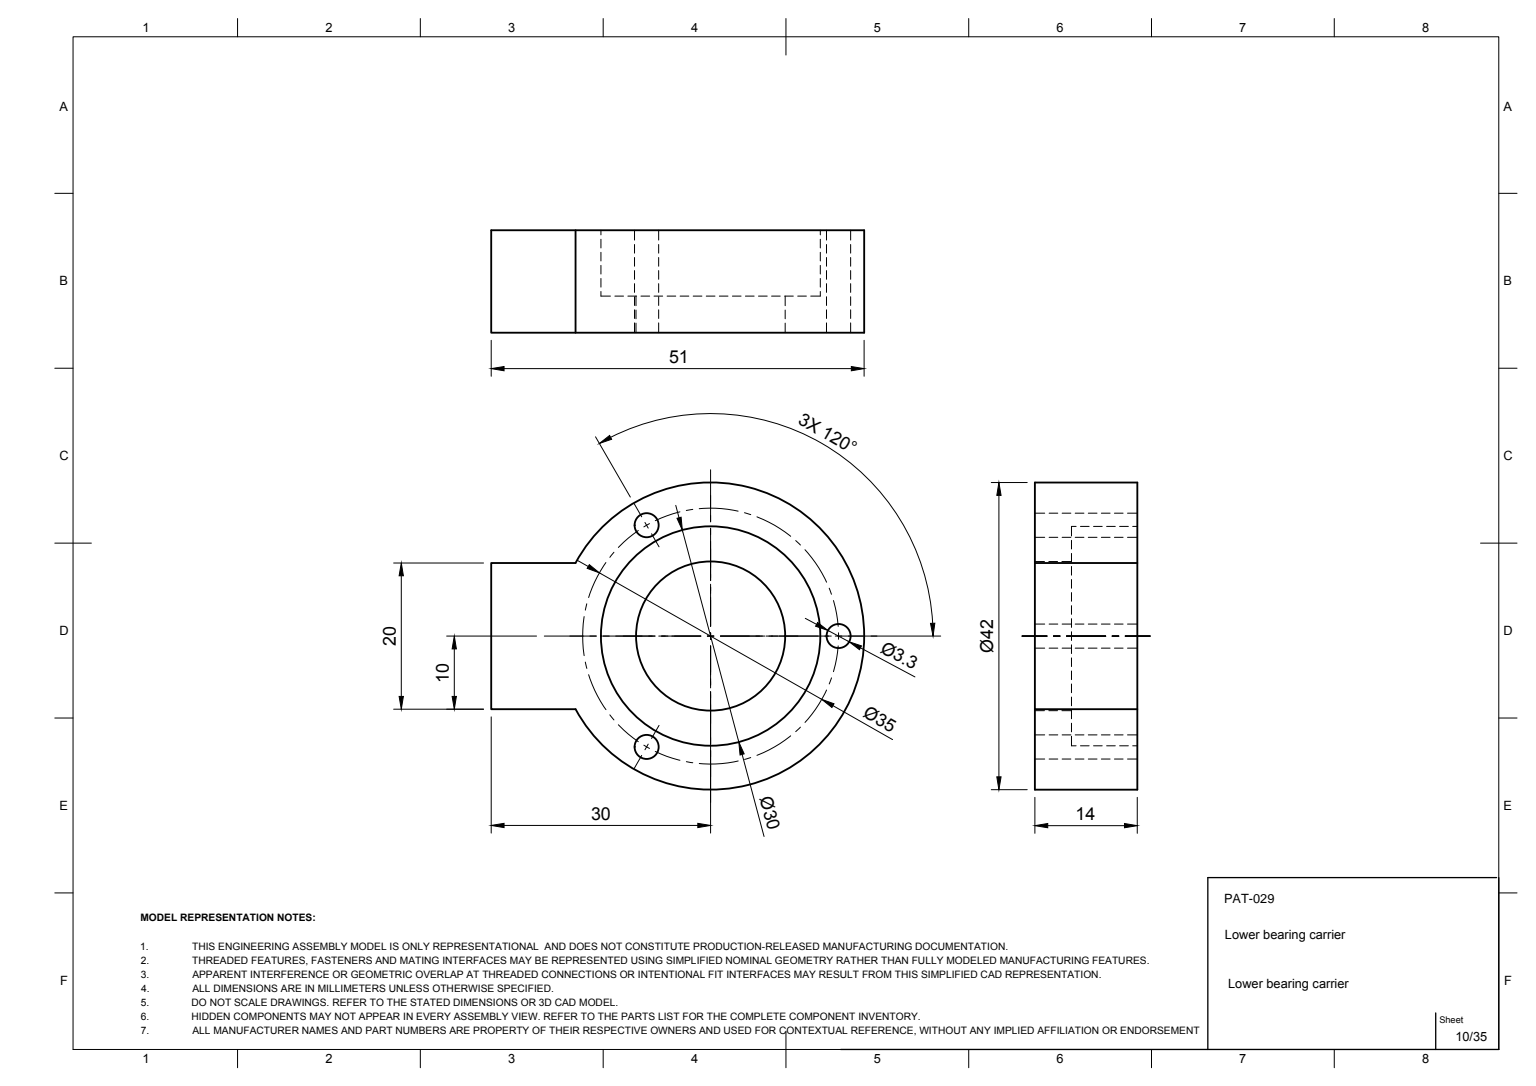
ISO-10303-21;
HEADER;
/* Generated by software containing ST-Developer
 * from STEP Tools, Inc. (www.steptools.com) 
 */

FILE_DESCRIPTION(
/* description */ ('Door-style hinge test fixture with detent'),
/* implementation_level */ '2;1');

FILE_NAME(
/* name */ 'Lower bearing carrier.step',
/* time_stamp */ '2026-10-28T03:24:57-07:00',
/* author */ (''),
/* organization */ (''),
/* preprocessor_version */ 'ST-DEVELOPER v20.2',
/* originating_system */ 'Autodesk Translation Framework v15.17.0.0',
/* authorisation */ '');

FILE_SCHEMA (('AUTOMOTIVE_DESIGN { 1 0 10303 214 3 1 1 }'));
ENDSEC;

DATA;
#10=MECHANICAL_DESIGN_GEOMETRIC_PRESENTATION_REPRESENTATION('',(#328),#9813);
#265=SHAPE_REPRESENTATION_RELATIONSHIP('SRR','None',#9942,#296);
#296=ADVANCED_BREP_SHAPE_REPRESENTATION('',(#368),#9785);
#328=STYLED_ITEM('',(#10183),#368);
#368=MANIFOLD_SOLID_BREP('Body1',#4759);
#423=FACE_BOUND('',#1025,.T.);
#424=FACE_BOUND('',#1028,.T.);
#425=FACE_BOUND('',#1029,.T.);
#426=FACE_BOUND('',#1030,.T.);
#427=FACE_BOUND('',#1031,.T.);
#428=FACE_BOUND('',#1037,.T.);
#429=FACE_BOUND('',#1038,.T.);
#430=FACE_BOUND('',#1039,.T.);
#431=FACE_BOUND('',#1040,.T.);
#536=PLANE('',#5230);
#537=PLANE('',#5234);
#538=PLANE('',#5236);
#539=PLANE('',#5237);
#540=PLANE('',#5238);
#541=PLANE('',#5241);
#711=FACE_OUTER_BOUND('',#1020,.T.);
#712=FACE_OUTER_BOUND('',#1021,.T.);
#713=FACE_OUTER_BOUND('',#1022,.T.);
#714=FACE_OUTER_BOUND('',#1023,.T.);
#715=FACE_OUTER_BOUND('',#1024,.T.);
#716=FACE_OUTER_BOUND('',#1026,.T.);
#717=FACE_OUTER_BOUND('',#1027,.T.);
#718=FACE_OUTER_BOUND('',#1032,.T.);
#719=FACE_OUTER_BOUND('',#1033,.T.);
#720=FACE_OUTER_BOUND('',#1034,.T.);
#721=FACE_OUTER_BOUND('',#1035,.T.);
#722=FACE_OUTER_BOUND('',#1036,.T.);
#1020=EDGE_LOOP('',(#3423,#3424,#3425,#3426));
#1021=EDGE_LOOP('',(#3427,#3428,#3429,#3430));
#1022=EDGE_LOOP('',(#3431,#3432,#3433,#3434));
#1023=EDGE_LOOP('',(#3435,#3436,#3437,#3438));
#1024=EDGE_LOOP('',(#3439));
#1025=EDGE_LOOP('',(#3440));
#1026=EDGE_LOOP('',(#3441,#3442,#3443,#3444));
#1027=EDGE_LOOP('',(#3445,#3446,#3447,#3448));
#1028=EDGE_LOOP('',(#3449));
#1029=EDGE_LOOP('',(#3450));
#1030=EDGE_LOOP('',(#3451));
#1031=EDGE_LOOP('',(#3452));
#1032=EDGE_LOOP('',(#3453,#3454,#3455,#3456));
#1033=EDGE_LOOP('',(#3457,#3458,#3459,#3460));
#1034=EDGE_LOOP('',(#3461,#3462,#3463,#3464));
#1035=EDGE_LOOP('',(#3465,#3466,#3467,#3468));
#1036=EDGE_LOOP('',(#3469,#3470,#3471,#3472));
#1037=EDGE_LOOP('',(#3473));
#1038=EDGE_LOOP('',(#3474));
#1039=EDGE_LOOP('',(#3475));
#1040=EDGE_LOOP('',(#3476));
#1418=LINE('',#7537,#1738);
#1419=LINE('',#7543,#1739);
#1420=LINE('',#7549,#1740);
#1421=LINE('',#7555,#1741);
#1422=LINE('',#7563,#1742);
#1423=LINE('',#7567,#1743);
#1424=LINE('',#7569,#1744);
#1425=LINE('',#7571,#1745);
#1426=LINE('',#7575,#1746);
#1427=LINE('',#7577,#1747);
#1428=LINE('',#7578,#1748);
#1429=LINE('',#7581,#1749);
#1430=LINE('',#7583,#1750);
#1431=LINE('',#7584,#1751);
#1432=LINE('',#7586,#1752);
#1738=VECTOR('',#5999,0.165);
#1739=VECTOR('',#6006,0.165);
#1740=VECTOR('',#6013,0.165);
#1741=VECTOR('',#6020,1.5);
#1742=VECTOR('',#6031,1.02);
#1743=VECTOR('',#6034,1.);
#1744=VECTOR('',#6035,1.);
#1745=VECTOR('',#6036,1.);
#1746=VECTOR('',#6041,1.);
#1747=VECTOR('',#6042,1.);
#1748=VECTOR('',#6043,1.);
#1749=VECTOR('',#6046,1.);
#1750=VECTOR('',#6047,1.);
#1751=VECTOR('',#6048,1.);
#1752=VECTOR('',#6051,1.);
#1998=CIRCLE('',#5219,0.165);
#1999=CIRCLE('',#5220,0.165);
#2000=CIRCLE('',#5222,0.165);
#2001=CIRCLE('',#5223,0.165);
#2002=CIRCLE('',#5225,0.165);
#2003=CIRCLE('',#5226,0.165);
#2004=CIRCLE('',#5228,1.5);
#2005=CIRCLE('',#5229,1.5);
#2006=CIRCLE('',#5231,1.02);
#2007=CIRCLE('',#5233,1.02);
#2008=CIRCLE('',#5235,2.1);
#2009=CIRCLE('',#5240,2.1);
#2293=VERTEX_POINT('',#7534);
#2294=VERTEX_POINT('',#7536);
#2295=VERTEX_POINT('',#7540);
#2296=VERTEX_POINT('',#7542);
#2297=VERTEX_POINT('',#7546);
#2298=VERTEX_POINT('',#7548);
#2299=VERTEX_POINT('',#7552);
#2300=VERTEX_POINT('',#7554);
#2301=VERTEX_POINT('',#7558);
#2302=VERTEX_POINT('',#7561);
#2303=VERTEX_POINT('',#7565);
#2304=VERTEX_POINT('',#7566);
#2305=VERTEX_POINT('',#7568);
#2306=VERTEX_POINT('',#7570);
#2307=VERTEX_POINT('',#7574);
#2308=VERTEX_POINT('',#7576);
#2309=VERTEX_POINT('',#7580);
#2310=VERTEX_POINT('',#7582);
#2728=EDGE_CURVE('',#2293,#2293,#1998,.T.);
#2729=EDGE_CURVE('',#2293,#2294,#1418,.T.);
#2730=EDGE_CURVE('',#2294,#2294,#1999,.T.);
#2731=EDGE_CURVE('',#2295,#2295,#2000,.T.);
#2732=EDGE_CURVE('',#2295,#2296,#1419,.T.);
#2733=EDGE_CURVE('',#2296,#2296,#2001,.T.);
#2734=EDGE_CURVE('',#2297,#2297,#2002,.T.);
#2735=EDGE_CURVE('',#2297,#2298,#1420,.T.);
#2736=EDGE_CURVE('',#2298,#2298,#2003,.T.);
#2737=EDGE_CURVE('',#2299,#2299,#2004,.T.);
#2738=EDGE_CURVE('',#2299,#2300,#1421,.T.);
#2739=EDGE_CURVE('',#2300,#2300,#2005,.T.);
#2740=EDGE_CURVE('',#2301,#2301,#2006,.T.);
#2741=EDGE_CURVE('',#2302,#2302,#2007,.T.);
#2742=EDGE_CURVE('',#2302,#2301,#1422,.T.);
#2743=EDGE_CURVE('',#2303,#2304,#1423,.T.);
#2744=EDGE_CURVE('',#2304,#2305,#1424,.T.);
#2745=EDGE_CURVE('',#2305,#2306,#1425,.T.);
#2746=EDGE_CURVE('',#2306,#2303,#2008,.T.);
#2747=EDGE_CURVE('',#2307,#2303,#1426,.T.);
#2748=EDGE_CURVE('',#2307,#2308,#1427,.T.);
#2749=EDGE_CURVE('',#2308,#2304,#1428,.T.);
#2750=EDGE_CURVE('',#2306,#2309,#1429,.T.);
#2751=EDGE_CURVE('',#2310,#2305,#1430,.T.);
#2752=EDGE_CURVE('',#2310,#2309,#1431,.T.);
#2753=EDGE_CURVE('',#2308,#2310,#1432,.T.);
#2754=EDGE_CURVE('',#2309,#2307,#2009,.T.);
#3423=ORIENTED_EDGE('',*,*,#2728,.F.);
#3424=ORIENTED_EDGE('',*,*,#2729,.T.);
#3425=ORIENTED_EDGE('',*,*,#2730,.F.);
#3426=ORIENTED_EDGE('',*,*,#2729,.F.);
#3427=ORIENTED_EDGE('',*,*,#2731,.F.);
#3428=ORIENTED_EDGE('',*,*,#2732,.T.);
#3429=ORIENTED_EDGE('',*,*,#2733,.F.);
#3430=ORIENTED_EDGE('',*,*,#2732,.F.);
#3431=ORIENTED_EDGE('',*,*,#2734,.F.);
#3432=ORIENTED_EDGE('',*,*,#2735,.T.);
#3433=ORIENTED_EDGE('',*,*,#2736,.F.);
#3434=ORIENTED_EDGE('',*,*,#2735,.F.);
#3435=ORIENTED_EDGE('',*,*,#2737,.F.);
#3436=ORIENTED_EDGE('',*,*,#2738,.T.);
#3437=ORIENTED_EDGE('',*,*,#2739,.F.);
#3438=ORIENTED_EDGE('',*,*,#2738,.F.);
#3439=ORIENTED_EDGE('',*,*,#2737,.T.);
#3440=ORIENTED_EDGE('',*,*,#2740,.F.);
#3441=ORIENTED_EDGE('',*,*,#2741,.F.);
#3442=ORIENTED_EDGE('',*,*,#2742,.T.);
#3443=ORIENTED_EDGE('',*,*,#2740,.T.);
#3444=ORIENTED_EDGE('',*,*,#2742,.F.);
#3445=ORIENTED_EDGE('',*,*,#2743,.T.);
#3446=ORIENTED_EDGE('',*,*,#2744,.T.);
#3447=ORIENTED_EDGE('',*,*,#2745,.T.);
#3448=ORIENTED_EDGE('',*,*,#2746,.T.);
#3449=ORIENTED_EDGE('',*,*,#2730,.T.);
#3450=ORIENTED_EDGE('',*,*,#2733,.T.);
#3451=ORIENTED_EDGE('',*,*,#2736,.T.);
#3452=ORIENTED_EDGE('',*,*,#2739,.T.);
#3453=ORIENTED_EDGE('',*,*,#2747,.F.);
#3454=ORIENTED_EDGE('',*,*,#2748,.T.);
#3455=ORIENTED_EDGE('',*,*,#2749,.T.);
#3456=ORIENTED_EDGE('',*,*,#2743,.F.);
#3457=ORIENTED_EDGE('',*,*,#2750,.F.);
#3458=ORIENTED_EDGE('',*,*,#2745,.F.);
#3459=ORIENTED_EDGE('',*,*,#2751,.F.);
#3460=ORIENTED_EDGE('',*,*,#2752,.T.);
#3461=ORIENTED_EDGE('',*,*,#2753,.T.);
#3462=ORIENTED_EDGE('',*,*,#2751,.T.);
#3463=ORIENTED_EDGE('',*,*,#2744,.F.);
#3464=ORIENTED_EDGE('',*,*,#2749,.F.);
#3465=ORIENTED_EDGE('',*,*,#2747,.T.);
#3466=ORIENTED_EDGE('',*,*,#2746,.F.);
#3467=ORIENTED_EDGE('',*,*,#2750,.T.);
#3468=ORIENTED_EDGE('',*,*,#2754,.T.);
#3469=ORIENTED_EDGE('',*,*,#2754,.F.);
#3470=ORIENTED_EDGE('',*,*,#2752,.F.);
#3471=ORIENTED_EDGE('',*,*,#2753,.F.);
#3472=ORIENTED_EDGE('',*,*,#2748,.F.);
#3473=ORIENTED_EDGE('',*,*,#2728,.T.);
#3474=ORIENTED_EDGE('',*,*,#2731,.T.);
#3475=ORIENTED_EDGE('',*,*,#2734,.T.);
#3476=ORIENTED_EDGE('',*,*,#2741,.T.);
#4393=CYLINDRICAL_SURFACE('',#5218,0.165);
#4394=CYLINDRICAL_SURFACE('',#5221,0.165);
#4395=CYLINDRICAL_SURFACE('',#5224,0.165);
#4396=CYLINDRICAL_SURFACE('',#5227,1.5);
#4397=CYLINDRICAL_SURFACE('',#5232,1.02);
#4398=CYLINDRICAL_SURFACE('',#5239,2.1);
#4516=ADVANCED_FACE('',(#711),#4393,.F.);
#4517=ADVANCED_FACE('',(#712),#4394,.F.);
#4518=ADVANCED_FACE('',(#713),#4395,.F.);
#4519=ADVANCED_FACE('',(#714),#4396,.F.);
#4520=ADVANCED_FACE('',(#715,#423),#536,.T.);
#4521=ADVANCED_FACE('',(#716),#4397,.F.);
#4522=ADVANCED_FACE('',(#717,#424,#425,#426,#427),#537,.T.);
#4523=ADVANCED_FACE('',(#718),#538,.T.);
#4524=ADVANCED_FACE('',(#719),#539,.T.);
#4525=ADVANCED_FACE('',(#720),#540,.T.);
#4526=ADVANCED_FACE('',(#721),#4398,.T.);
#4527=ADVANCED_FACE('',(#722,#428,#429,#430,#431),#541,.F.);
#4759=CLOSED_SHELL('',(#4516,#4517,#4518,#4519,#4520,#4521,#4522,#4523,
#4524,#4525,#4526,#4527));
#5217=AXIS2_PLACEMENT_3D('',#7532,#5993,#5994);
#5218=AXIS2_PLACEMENT_3D('',#7533,#5995,#5996);
#5219=AXIS2_PLACEMENT_3D('',#7535,#5997,#5998);
#5220=AXIS2_PLACEMENT_3D('',#7538,#6000,#6001);
#5221=AXIS2_PLACEMENT_3D('',#7539,#6002,#6003);
#5222=AXIS2_PLACEMENT_3D('',#7541,#6004,#6005);
#5223=AXIS2_PLACEMENT_3D('',#7544,#6007,#6008);
#5224=AXIS2_PLACEMENT_3D('',#7545,#6009,#6010);
#5225=AXIS2_PLACEMENT_3D('',#7547,#6011,#6012);
#5226=AXIS2_PLACEMENT_3D('',#7550,#6014,#6015);
#5227=AXIS2_PLACEMENT_3D('',#7551,#6016,#6017);
#5228=AXIS2_PLACEMENT_3D('',#7553,#6018,#6019);
#5229=AXIS2_PLACEMENT_3D('',#7556,#6021,#6022);
#5230=AXIS2_PLACEMENT_3D('',#7557,#6023,#6024);
#5231=AXIS2_PLACEMENT_3D('',#7559,#6025,#6026);
#5232=AXIS2_PLACEMENT_3D('',#7560,#6027,#6028);
#5233=AXIS2_PLACEMENT_3D('',#7562,#6029,#6030);
#5234=AXIS2_PLACEMENT_3D('',#7564,#6032,#6033);
#5235=AXIS2_PLACEMENT_3D('',#7572,#6037,#6038);
#5236=AXIS2_PLACEMENT_3D('',#7573,#6039,#6040);
#5237=AXIS2_PLACEMENT_3D('',#7579,#6044,#6045);
#5238=AXIS2_PLACEMENT_3D('',#7585,#6049,#6050);
#5239=AXIS2_PLACEMENT_3D('',#7587,#6052,#6053);
#5240=AXIS2_PLACEMENT_3D('',#7588,#6054,#6055);
#5241=AXIS2_PLACEMENT_3D('',#7589,#6056,#6057);
#5993=DIRECTION('axis',(0.,0.,1.));
#5994=DIRECTION('refdir',(1.,0.,0.));
#5995=DIRECTION('center_axis',(0.,0.,1.));
#5996=DIRECTION('ref_axis',(1.,0.,0.));
#5997=DIRECTION('center_axis',(0.,0.,1.));
#5998=DIRECTION('ref_axis',(1.,0.,0.));
#5999=DIRECTION('',(0.,0.,1.));
#6000=DIRECTION('center_axis',(0.,0.,-1.));
#6001=DIRECTION('ref_axis',(1.,0.,0.));
#6002=DIRECTION('center_axis',(0.,0.,1.));
#6003=DIRECTION('ref_axis',(1.,0.,0.));
#6004=DIRECTION('center_axis',(0.,0.,1.));
#6005=DIRECTION('ref_axis',(1.,0.,0.));
#6006=DIRECTION('',(0.,0.,1.));
#6007=DIRECTION('center_axis',(0.,0.,-1.));
#6008=DIRECTION('ref_axis',(1.,0.,0.));
#6009=DIRECTION('center_axis',(0.,0.,1.));
#6010=DIRECTION('ref_axis',(1.,0.,0.));
#6011=DIRECTION('center_axis',(0.,0.,1.));
#6012=DIRECTION('ref_axis',(1.,0.,0.));
#6013=DIRECTION('',(0.,0.,1.));
#6014=DIRECTION('center_axis',(0.,0.,-1.));
#6015=DIRECTION('ref_axis',(1.,0.,0.));
#6016=DIRECTION('center_axis',(0.,0.,1.));
#6017=DIRECTION('ref_axis',(1.,0.,0.));
#6018=DIRECTION('center_axis',(0.,0.,1.));
#6019=DIRECTION('ref_axis',(1.,0.,0.));
#6020=DIRECTION('',(0.,0.,1.));
#6021=DIRECTION('center_axis',(0.,0.,-1.));
#6022=DIRECTION('ref_axis',(1.,0.,0.));
#6023=DIRECTION('center_axis',(0.,0.,1.));
#6024=DIRECTION('ref_axis',(1.,0.,0.));
#6025=DIRECTION('center_axis',(0.,0.,1.));
#6026=DIRECTION('ref_axis',(1.,0.,0.));
#6027=DIRECTION('center_axis',(0.,0.,1.));
#6028=DIRECTION('ref_axis',(1.,0.,0.));
#6029=DIRECTION('center_axis',(0.,0.,1.));
#6030=DIRECTION('ref_axis',(1.,0.,0.));
#6031=DIRECTION('',(0.,0.,1.));
#6032=DIRECTION('center_axis',(0.,0.,1.));
#6033=DIRECTION('ref_axis',(1.,0.,0.));
#6034=DIRECTION('',(-1.,0.,0.));
#6035=DIRECTION('',(0.,-1.,0.));
#6036=DIRECTION('',(1.,0.,0.));
#6037=DIRECTION('center_axis',(0.,0.,1.));
#6038=DIRECTION('ref_axis',(1.,0.,0.));
#6039=DIRECTION('center_axis',(0.,1.,0.));
#6040=DIRECTION('ref_axis',(-1.,0.,0.));
#6041=DIRECTION('',(0.,0.,1.));
#6042=DIRECTION('',(-1.,0.,0.));
#6043=DIRECTION('',(0.,0.,1.));
#6044=DIRECTION('center_axis',(0.,-1.,0.));
#6045=DIRECTION('ref_axis',(1.,0.,0.));
#6046=DIRECTION('',(0.,0.,-1.));
#6047=DIRECTION('',(0.,0.,1.));
#6048=DIRECTION('',(1.,0.,0.));
#6049=DIRECTION('center_axis',(-1.,0.,0.));
#6050=DIRECTION('ref_axis',(0.,-1.,0.));
#6051=DIRECTION('',(0.,-1.,0.));
#6052=DIRECTION('center_axis',(0.,0.,1.));
#6053=DIRECTION('ref_axis',(1.,0.,0.));
#6054=DIRECTION('center_axis',(0.,0.,1.));
#6055=DIRECTION('ref_axis',(1.,0.,0.));
#6056=DIRECTION('center_axis',(0.,0.,1.));
#6057=DIRECTION('ref_axis',(1.,0.,0.));
#7532=CARTESIAN_POINT('',(0.,0.,0.));
#7533=CARTESIAN_POINT('Origin',(1.75,0.,1.9));
#7534=CARTESIAN_POINT('',(1.585,-2.02066721859313E-17,2.));
#7535=CARTESIAN_POINT('Origin',(1.75,0.,2.));
#7536=CARTESIAN_POINT('',(1.585,2.02066721859313E-17,3.4));
#7537=CARTESIAN_POINT('',(1.585,-2.02066721859313E-17,1.9));
#7538=CARTESIAN_POINT('Origin',(1.75,0.,3.4));
#7539=CARTESIAN_POINT('Origin',(-0.875,1.51554445662277,1.9));
#7540=CARTESIAN_POINT('',(-1.04,1.51554445662277,2.));
#7541=CARTESIAN_POINT('Origin',(-0.875,1.51554445662277,2.));
#7542=CARTESIAN_POINT('',(-1.04,1.51554445662277,3.4));
#7543=CARTESIAN_POINT('',(-1.04,1.51554445662277,1.9));
#7544=CARTESIAN_POINT('Origin',(-0.875,1.51554445662277,3.4));
#7545=CARTESIAN_POINT('Origin',(-0.875000000000001,-1.51554445662277,1.9));
#7546=CARTESIAN_POINT('',(-1.04,-1.51554445662277,2.));
#7547=CARTESIAN_POINT('Origin',(-0.875000000000001,-1.51554445662277,2.));
#7548=CARTESIAN_POINT('',(-1.04,-1.51554445662277,3.4));
#7549=CARTESIAN_POINT('',(-1.04,-1.51554445662277,1.9));
#7550=CARTESIAN_POINT('Origin',(-0.875000000000001,-1.51554445662277,3.4));
#7551=CARTESIAN_POINT('Origin',(0.,0.,2.5));
#7552=CARTESIAN_POINT('',(-1.5,-1.83697019872103E-16,2.5));
#7553=CARTESIAN_POINT('Origin',(0.,0.,2.5));
#7554=CARTESIAN_POINT('',(-1.5,1.83697019872103E-16,3.4));
#7555=CARTESIAN_POINT('',(-1.5,-1.83697019872103E-16,2.5));
#7556=CARTESIAN_POINT('Origin',(0.,0.,3.4));
#7557=CARTESIAN_POINT('Origin',(0.,0.,2.5));
#7558=CARTESIAN_POINT('',(-1.02,-1.2491397351303E-16,2.5));
#7559=CARTESIAN_POINT('Origin',(0.,0.,2.5));
#7560=CARTESIAN_POINT('Origin',(0.,0.,1.9));
#7561=CARTESIAN_POINT('',(-1.02,-1.2491397351303E-16,2.));
#7562=CARTESIAN_POINT('Origin',(0.,0.,2.));
#7563=CARTESIAN_POINT('',(-1.02,-1.2491397351303E-16,1.9));
#7564=CARTESIAN_POINT('Origin',(0.,0.,3.4));
#7565=CARTESIAN_POINT('',(-1.84661853126194,1.,3.4));
#7566=CARTESIAN_POINT('',(-3.,1.,3.4));
#7567=CARTESIAN_POINT('',(0.,1.,3.4));
#7568=CARTESIAN_POINT('',(-3.,-1.,3.4));
#7569=CARTESIAN_POINT('',(-3.,1.,3.4));
#7570=CARTESIAN_POINT('',(-1.84661853126194,-1.,3.4));
#7571=CARTESIAN_POINT('',(-3.,-1.,3.4));
#7572=CARTESIAN_POINT('Origin',(0.,0.,3.4));
#7573=CARTESIAN_POINT('Origin',(0.,1.,2.));
#7574=CARTESIAN_POINT('',(-1.84661853126194,1.,2.));
#7575=CARTESIAN_POINT('',(-1.84661853126194,1.,2.));
#7576=CARTESIAN_POINT('',(-3.,1.,2.));
#7577=CARTESIAN_POINT('',(0.,1.,2.));
#7578=CARTESIAN_POINT('',(-3.,1.,2.));
#7579=CARTESIAN_POINT('Origin',(-3.,-1.,2.));
#7580=CARTESIAN_POINT('',(-1.84661853126194,-1.,2.));
#7581=CARTESIAN_POINT('',(-1.84661853126194,-1.,2.));
#7582=CARTESIAN_POINT('',(-3.,-1.,2.));
#7583=CARTESIAN_POINT('',(-3.,-1.,2.));
#7584=CARTESIAN_POINT('',(-3.,-1.,2.));
#7585=CARTESIAN_POINT('Origin',(-3.,1.,2.));
#7586=CARTESIAN_POINT('',(-3.,1.,2.));
#7587=CARTESIAN_POINT('Origin',(0.,0.,2.));
#7588=CARTESIAN_POINT('Origin',(0.,0.,2.));
#7589=CARTESIAN_POINT('Origin',(0.,0.,2.));
#9749=UNCERTAINTY_MEASURE_WITH_UNIT(LENGTH_MEASURE(0.001),#9814,
'DISTANCE_ACCURACY_VALUE',
'Maximum model space distance between geometric entities at asserted c
onnectivities');
#9777=UNCERTAINTY_MEASURE_WITH_UNIT(LENGTH_MEASURE(0.001),#9814,
'DISTANCE_ACCURACY_VALUE',
'Maximum model space distance between geometric entities at asserted c
onnectivities');
#9785=(
GEOMETRIC_REPRESENTATION_CONTEXT(3)
GLOBAL_UNCERTAINTY_ASSIGNED_CONTEXT((#9749))
GLOBAL_UNIT_ASSIGNED_CONTEXT((#9814,#9816,#9817))
REPRESENTATION_CONTEXT('','3D')
);
#9813=(
GEOMETRIC_REPRESENTATION_CONTEXT(3)
GLOBAL_UNCERTAINTY_ASSIGNED_CONTEXT((#9777))
GLOBAL_UNIT_ASSIGNED_CONTEXT((#9814,#9816,#9817))
REPRESENTATION_CONTEXT('','3D')
);
#9814=(
LENGTH_UNIT()
NAMED_UNIT(*)
SI_UNIT(.CENTI.,.METRE.)
);
#9816=(
NAMED_UNIT(*)
PLANE_ANGLE_UNIT()
SI_UNIT($,.RADIAN.)
);
#9817=(
NAMED_UNIT(*)
SI_UNIT($,.STERADIAN.)
SOLID_ANGLE_UNIT()
);
#9825=SHAPE_DEFINITION_REPRESENTATION(#9860,#9942);
#9860=PRODUCT_DEFINITION_SHAPE('',$,#9978);
#9942=SHAPE_REPRESENTATION('',(#5217),#9785);
#9970=PRODUCT_DEFINITION_CONTEXT('part definition',#10077,'design');
#9978=PRODUCT_DEFINITION('Lower bearing carrier',
'Lower bearing carrier',#10013,#9970);
#10013=PRODUCT_DEFINITION_FORMATION('',$,#10086);
#10077=APPLICATION_CONTEXT(
'Core Data for Automotive Mechanical Design Process');
#10078=PRODUCT_CONTEXT('part definition',#10077,'mechanical');
#10086=PRODUCT('Lower bearing carrier','Lower bearing carrier',
'Lower bearing carrier',(#10078));
#10177=COLOUR_RGB('Grey',0.48,0.52,0.57);
#10178=FILL_AREA_STYLE_COLOUR('',#10177);
#10179=FILL_AREA_STYLE('',(#10178));
#10180=SURFACE_STYLE_FILL_AREA(#10179);
#10181=SURFACE_SIDE_STYLE('',(#10180));
#10182=SURFACE_STYLE_USAGE(.BOTH.,#10181);
#10183=PRESENTATION_STYLE_ASSIGNMENT((#10182));
ENDSEC;
END-ISO-10303-21;
